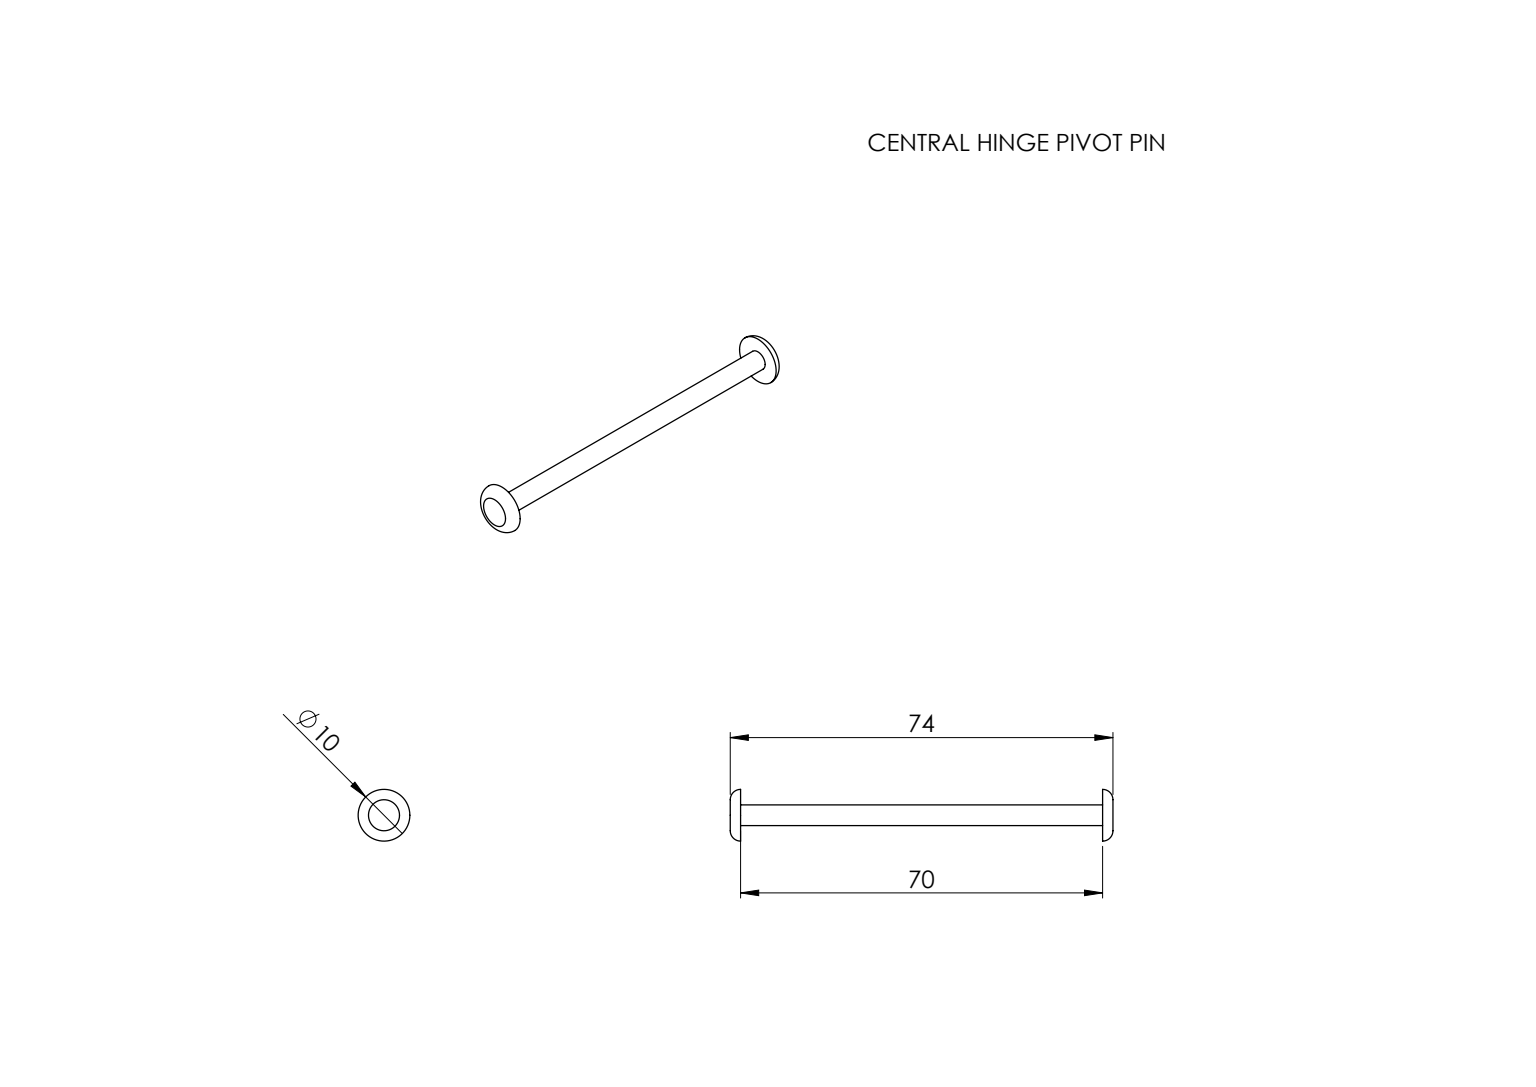
ISO-10303-21;
HEADER;
FILE_DESCRIPTION (('STEP AP214'),
    '1' );
FILE_NAME ('Central Hinge Pivot Pin.step',
    '2026-10-02T13:02:33',
    ( '' ),
    ( '' ),
    'SwSTEP 2.0',
    'SolidWorks 2026',
    '' );
FILE_SCHEMA (( 'AUTOMOTIVE_DESIGN' ));
ENDSEC;

DATA;
#71=CIRCLE ( 'NONE', #9451, 3.000000000000000000 ) ;
#84=CARTESIAN_POINT ( 'NONE',  ( 0.000000000000000000, 0.000000000000000000, 35.00000000000000000 ) ) ;
#87=( GEOMETRIC_REPRESENTATION_CONTEXT ( 3 ) GLOBAL_UNCERTAINTY_ASSIGNED_CONTEXT ( ( #8912 ) ) GLOBAL_UNIT_ASSIGNED_CONTEXT ( ( #3872, #4067, #6666 ) ) REPRESENTATION_CONTEXT ( 'NONE', 'WORKASPACE' ) );
#156=EDGE_LOOP ( 'NONE', ( #2014, #11521, #8711, #17506 ) ) ;
#171=FACE_OUTER_BOUND ( 'NONE', #4320, .T. ) ;
#180=ORIENTED_EDGE ( 'NONE', *, *, #16256, .T. ) ;
#259=DIRECTION ( 'NONE',  ( 1.000000000000000000, 0.000000000000000000, -0.000000000000000000 ) ) ;
#293=DIRECTION ( 'NONE',  ( -1.000000000000000000, 0.000000000000000000, 0.000000000000000000 ) ) ;
#355=CIRCLE ( 'NONE', #13059, 2.000000000000000000 ) ;
#373=ORIENTED_EDGE ( 'NONE', *, *, #11541, .F. ) ;
#379=ORIENTED_EDGE ( 'NONE', *, *, #9515, .T. ) ;
#388=STYLED_ITEM ( 'NONE', ( #17094 ), #8708 ) ;
#454=PRODUCT ( 'Central Hinge Pivot Pin', 'Central Hinge Pivot Pin', '', ( #9983 ) ) ;
#476=CARTESIAN_POINT ( 'NONE',  ( 3.000000000000000000, 4.898587196589412829E-16, -37.00000000000000711 ) ) ;
#676=CARTESIAN_POINT ( 'NONE',  ( 0.000000000000000000, 0.000000000000000000, 35.00000000000000000 ) ) ;
#732=CARTESIAN_POINT ( 'NONE',  ( 0.000000000000000000, 0.000000000000000000, -35.00000000000000000 ) ) ;
#784=SURFACE_SIDE_STYLE ('',( #16717 ) ) ;
#816=DIRECTION ( 'NONE',  ( 0.000000000000000000, 0.000000000000000000, 1.000000000000000000 ) ) ;
#899=DIRECTION ( 'NONE',  ( 0.000000000000000000, 0.000000000000000000, -1.000000000000000000 ) ) ;
#927=ADVANCED_FACE ( 'NONE', ( #17116 ), #14530, .T. ) ;
#967=CIRCLE ( 'NONE', #3346, 2.000000000000001776 ) ;
#1020=DIRECTION ( 'NONE',  ( -0.000000000000000000, -0.000000000000000000, -1.000000000000000000 ) ) ;
#1061=ORIENTED_EDGE ( 'NONE', *, *, #6669, .F. ) ;
#1218=FACE_OUTER_BOUND ( 'NONE', #3277, .T. ) ;
#1275=ORIENTED_EDGE ( 'NONE', *, *, #17968, .T. ) ;
#1295=DIRECTION ( 'NONE',  ( 1.000000000000000000, 0.000000000000000000, 0.000000000000000000 ) ) ;
#1354=CARTESIAN_POINT ( 'NONE',  ( 0.000000000000000000, 0.000000000000000000, -35.00000000000000000 ) ) ;
#1762=DIRECTION ( 'NONE',  ( 1.000000000000000000, 0.000000000000000000, 0.000000000000000000 ) ) ;
#1884=FACE_OUTER_BOUND ( 'NONE', #16108, .T. ) ;
#1930=EDGE_LOOP ( 'NONE', ( #9001, #9036, #2188, #4675 ) ) ;
#1944=PRESENTATION_STYLE_ASSIGNMENT (( #8874 ) ) ;
#1972=EDGE_LOOP ( 'NONE', ( #15195, #7068 ) ) ;
#1996=FACE_OUTER_BOUND ( 'NONE', #18432, .T. ) ;
#2014=ORIENTED_EDGE ( 'NONE', *, *, #11541, .T. ) ;
#2065=DIRECTION ( 'NONE',  ( 1.000000000000000000, 0.000000000000000000, 0.000000000000000000 ) ) ;
#2110=PRODUCT_DEFINITION ( 'UNKNOWN', '', #18444, #16492 ) ;
#2188=ORIENTED_EDGE ( 'NONE', *, *, #15045, .F. ) ;
#2222=DIRECTION ( 'NONE',  ( 1.000000000000000000, 0.000000000000000000, 0.000000000000000000 ) ) ;
#2273=ORIENTED_EDGE ( 'NONE', *, *, #3881, .T. ) ;
#2347=ORIENTED_EDGE ( 'NONE', *, *, #17236, .F. ) ;
#2378=TOROIDAL_SURFACE ( 'NONE', #5096, 3.000000000000000000, 2.000000000000000000 ) ;
#2422=CIRCLE ( 'NONE', #13007, 5.000000000000000000 ) ;
#2462=EDGE_CURVE ( 'NONE', #8941, #8532, #71, .T. ) ;
#2485=LINE ( 'NONE', #15360, #17967 ) ;
#2610=DIRECTION ( 'NONE',  ( 1.000000000000000000, 0.000000000000000000, 0.000000000000000000 ) ) ;
#2638=FACE_OUTER_BOUND ( 'NONE', #10893, .T. ) ;
#2654=VERTEX_POINT ( 'NONE', #9678 ) ;
#2742=DIRECTION ( 'NONE',  ( 0.000000000000000000, 0.000000000000000000, 1.000000000000000000 ) ) ;
#2755=DIRECTION ( 'NONE',  ( 0.000000000000000000, 0.000000000000000000, 1.000000000000000000 ) ) ;
#3019=ADVANCED_FACE ( 'NONE', ( #4031 ), #15601, .T. ) ;
#3081=FILL_AREA_STYLE_COLOUR ( '', #13822 ) ;
#3129=DIRECTION ( 'NONE',  ( -1.000000000000000000, 0.000000000000000000, 0.000000000000000000 ) ) ;
#3253=( NAMED_UNIT ( * ) PLANE_ANGLE_UNIT ( ) SI_UNIT ( $, .RADIAN. ) );
#3271=CIRCLE ( 'NONE', #10551, 3.000000000000000000 ) ;
#3277=EDGE_LOOP ( 'NONE', ( #2347, #7274, #18296, #12313 ) ) ;
#3346=AXIS2_PLACEMENT_3D ( 'NONE', #12462, #6513, #8306 ) ;
#3434=ADVANCED_FACE ( 'NONE', ( #7901 ), #10506, .T. ) ;
#3547=DIRECTION ( 'NONE',  ( 0.000000000000000000, 0.000000000000000000, -1.000000000000000000 ) ) ;
#3744=DIRECTION ( 'NONE',  ( 0.000000000000000000, 0.000000000000000000, 1.000000000000000000 ) ) ;
#3838=VERTEX_POINT ( 'NONE', #9282 ) ;
#3872=( LENGTH_UNIT ( ) NAMED_UNIT ( * ) SI_UNIT ( .MILLI., .METRE. ) );
#3874=CIRCLE ( 'NONE', #16614, 2.000000000000000000 ) ;
#3881=EDGE_CURVE ( 'NONE', #10603, #16711, #2422, .T. ) ;
#3973=DIRECTION ( 'NONE',  ( 1.000000000000000000, 0.000000000000000000, 0.000000000000000000 ) ) ;
#4031=FACE_OUTER_BOUND ( 'NONE', #14769, .T. ) ;
#4036=VERTEX_POINT ( 'NONE', #14821 ) ;
#4067=( NAMED_UNIT ( * ) PLANE_ANGLE_UNIT ( ) SI_UNIT ( $, .RADIAN. ) );
#4096=CARTESIAN_POINT ( 'NONE',  ( 0.000000000000000000, 0.000000000000000000, 35.00000000000000000 ) ) ;
#4141=PLANE ( 'NONE',  #5570 ) ;
#4183=DIRECTION ( 'NONE',  ( -1.000000000000000000, 1.224646799147353207E-16, 0.000000000000000000 ) ) ;
#4256=AXIS2_PLACEMENT_3D ( 'NONE', #732, #8958, #16371 ) ;
#4313=DIRECTION ( 'NONE',  ( 0.000000000000000000, 0.000000000000000000, 1.000000000000000000 ) ) ;
#4320=EDGE_LOOP ( 'NONE', ( #4636, #8294 ) ) ;
#4452=( GEOMETRIC_REPRESENTATION_CONTEXT ( 3 ) GLOBAL_UNCERTAINTY_ASSIGNED_CONTEXT ( ( #5444 ) ) GLOBAL_UNIT_ASSIGNED_CONTEXT ( ( #4502, #6419, #10283 ) ) REPRESENTATION_CONTEXT ( 'NONE', 'WORKASPACE' ) );
#4502=( LENGTH_UNIT ( ) NAMED_UNIT ( * ) SI_UNIT ( .MILLI., .METRE. ) );
#4516=EDGE_CURVE ( 'NONE', #10603, #8941, #8765, .T. ) ;
#4561=DIRECTION ( 'NONE',  ( 0.000000000000000000, 0.000000000000000000, -1.000000000000000000 ) ) ;
#4605=FACE_BOUND ( 'NONE', #1972, .T. ) ;
#4628=ORIENTED_EDGE ( 'NONE', *, *, #9298, .F. ) ;
#4636=ORIENTED_EDGE ( 'NONE', *, *, #8156, .F. ) ;
#4675=ORIENTED_EDGE ( 'NONE', *, *, #16432, .F. ) ;
#4681=ORIENTED_EDGE ( 'NONE', *, *, #10044, .F. ) ;
#4787=AXIS2_PLACEMENT_3D ( 'NONE', #15207, #1020, #2222 ) ;
#4803=ADVANCED_FACE ( 'NONE', ( #11642 ), #12064, .T. ) ;
#5007=ADVANCED_FACE ( 'NONE', ( #1884 ), #6066, .T. ) ;
#5024=CARTESIAN_POINT ( 'NONE',  ( 5.000000000000000000, 0.000000000000000000, 35.00000000000000000 ) ) ;
#5054=CIRCLE ( 'NONE', #17804, 2.000000000000000000 ) ;
#5071=CARTESIAN_POINT ( 'NONE',  ( 0.000000000000000000, 0.000000000000000000, -35.00000000000000000 ) ) ;
#5096=AXIS2_PLACEMENT_3D ( 'NONE', #7416, #10519, #6283 ) ;
#5163=CIRCLE ( 'NONE', #18227, 5.000000000000000000 ) ;
#5180=EDGE_LOOP ( 'NONE', ( #373, #17700 ) ) ;
#5261=CIRCLE ( 'NONE', #10986, 2.000000000000001776 ) ;
#5373=CARTESIAN_POINT ( 'NONE',  ( -3.000000000000000000, 0.000000000000000000, -37.00000000000000711 ) ) ;
#5444=UNCERTAINTY_MEASURE_WITH_UNIT (LENGTH_MEASURE( 1.000000000000000082E-05 ), #4502, 'distance_accuracy_value', 'NONE');
#5447=AXIS2_PLACEMENT_3D ( 'NONE', #4096, #8485, #1295 ) ;
#5570=AXIS2_PLACEMENT_3D ( 'NONE', #18529, #17077, #9846 ) ;
#5766=DIRECTION ( 'NONE',  ( -1.224646799147353207E-16, 1.000000000000000000, 0.000000000000000000 ) ) ;
#5851=DIRECTION ( 'NONE',  ( -1.000000000000000000, -1.224646799147353207E-16, 0.000000000000000000 ) ) ;
#5887=DIRECTION ( 'NONE',  ( -0.000000000000000000, -0.000000000000000000, -1.000000000000000000 ) ) ;
#5951=DIRECTION ( 'NONE',  ( 0.000000000000000000, 0.000000000000000000, 1.000000000000000000 ) ) ;
#6029=CLOSED_SHELL ( 'NONE', ( #3434, #4803, #5007, #7101, #3019, #9319, #9262, #16192, #17067, #927 ) ) ;
#6066=CYLINDRICAL_SURFACE ( 'NONE', #18164, 2.000000000000000000 ) ;
#6198=VERTEX_POINT ( 'NONE', #15959 ) ;
#6246=VERTEX_POINT ( 'NONE', #10038 ) ;
#6283=DIRECTION ( 'NONE',  ( -1.000000000000000000, 0.000000000000000000, 0.000000000000000000 ) ) ;
#6307=ORIENTED_EDGE ( 'NONE', *, *, #4516, .F. ) ;
#6419=( NAMED_UNIT ( * ) PLANE_ANGLE_UNIT ( ) SI_UNIT ( $, .RADIAN. ) );
#6513=DIRECTION ( 'NONE',  ( 0.000000000000000000, -1.000000000000000000, 0.000000000000000000 ) ) ;
#6666=( NAMED_UNIT ( * ) SI_UNIT ( $, .STERADIAN. ) SOLID_ANGLE_UNIT ( ) );
#6669=EDGE_CURVE ( 'NONE', #7437, #4036, #13199, .T. ) ;
#6721=DIRECTION ( 'NONE',  ( 0.000000000000000000, 0.000000000000000000, -1.000000000000000000 ) ) ;
#6821=ORIENTED_EDGE ( 'NONE', *, *, #16993, .F. ) ;
#6967=DIRECTION ( 'NONE',  ( 1.224646799147353207E-16, 1.000000000000000000, -0.000000000000000000 ) ) ;
#7068=ORIENTED_EDGE ( 'NONE', *, *, #6669, .T. ) ;
#7101=ADVANCED_FACE ( 'NONE', ( #1218 ), #11226, .T. ) ;
#7146=CARTESIAN_POINT ( 'NONE',  ( 0.000000000000000000, 0.000000000000000000, -35.00000000000000000 ) ) ;
#7274=ORIENTED_EDGE ( 'NONE', *, *, #11042, .F. ) ;
#7416=CARTESIAN_POINT ( 'NONE',  ( 0.000000000000000000, 0.000000000000000000, -35.00000000000000000 ) ) ;
#7437=VERTEX_POINT ( 'NONE', #9607 ) ;
#7451=FILL_AREA_STYLE ('',( #3081 ) ) ;
#7469=FACE_BOUND ( 'NONE', #13105, .T. ) ;
#7473=DIRECTION ( 'NONE',  ( 0.000000000000000000, 0.000000000000000000, 1.000000000000000000 ) ) ;
#7496=MECHANICAL_DESIGN_GEOMETRIC_PRESENTATION_REPRESENTATION('',(#16262),#18733);
#7542=( NAMED_UNIT ( * ) SI_UNIT ( $, .STERADIAN. ) SOLID_ANGLE_UNIT ( ) );
#7646=SURFACE_STYLE_FILL_AREA ( #7451 ) ;
#7728=SHAPE_REPRESENTATION_RELATIONSHIP ( 'NONE' , 'NONE' ,  #13127, #14079 ) ;
#7901=FACE_OUTER_BOUND ( 'NONE', #1930, .T. ) ;
#8156=EDGE_CURVE ( 'NONE', #13974, #2654, #14279, .T. ) ;
#8163=AXIS2_PLACEMENT_3D ( 'NONE', #11505, #5766, #5851 ) ;
#8274=SURFACE_STYLE_USAGE ( .BOTH. , #784 ) ;
#8294=ORIENTED_EDGE ( 'NONE', *, *, #16256, .F. ) ;
#8306=DIRECTION ( 'NONE',  ( 0.000000000000000000, 0.000000000000000000, -1.000000000000000000 ) ) ;
#8485=DIRECTION ( 'NONE',  ( 0.000000000000000000, 0.000000000000000000, 1.000000000000000000 ) ) ;
#8532=VERTEX_POINT ( 'NONE', #5373 ) ;
#8535=DIRECTION ( 'NONE',  ( 1.000000000000000000, 0.000000000000000000, 0.000000000000000000 ) ) ;
#8591=AXIS2_PLACEMENT_3D ( 'NONE', #15717, #2742, #8535 ) ;
#8696=EDGE_CURVE ( 'NONE', #4036, #3838, #2485, .T. ) ;
#8708=MANIFOLD_SOLID_BREP ( 'Fillet1', #6029 ) ;
#8711=ORIENTED_EDGE ( 'NONE', *, *, #16898, .F. ) ;
#8765=CIRCLE ( 'NONE', #8163, 2.000000000000000000 ) ;
#8792=DIRECTION ( 'NONE',  ( 1.000000000000000000, 0.000000000000000000, 0.000000000000000000 ) ) ;
#8874=SURFACE_STYLE_USAGE ( .BOTH. , #13583 ) ;
#8912=UNCERTAINTY_MEASURE_WITH_UNIT (LENGTH_MEASURE( 1.000000000000000082E-05 ), #3872, 'distance_accuracy_value', 'NONE');
#8941=VERTEX_POINT ( 'NONE', #476 ) ;
#8958=DIRECTION ( 'NONE',  ( 0.000000000000000000, 0.000000000000000000, -1.000000000000000000 ) ) ;
#9001=ORIENTED_EDGE ( 'NONE', *, *, #8156, .T. ) ;
#9036=ORIENTED_EDGE ( 'NONE', *, *, #16993, .T. ) ;
#9262=ADVANCED_FACE ( 'NONE', ( #2638 ), #4141, .T. ) ;
#9282=CARTESIAN_POINT ( 'NONE',  ( 2.000000000000000000, 0.000000000000000000, 35.00000000000000000 ) ) ;
#9298=EDGE_CURVE ( 'NONE', #13520, #6246, #15842, .T. ) ;
#9319=ADVANCED_FACE ( 'NONE', ( #7469, #171 ), #10581, .F. ) ;
#9395=DIRECTION ( 'NONE',  ( 0.000000000000000000, 0.000000000000000000, 1.000000000000000000 ) ) ;
#9451=AXIS2_PLACEMENT_3D ( 'NONE', #13259, #10141, #293 ) ;
#9515=EDGE_CURVE ( 'NONE', #16711, #8532, #5261, .T. ) ;
#9582=DIRECTION ( 'NONE',  ( 0.000000000000000000, 0.000000000000000000, 1.000000000000000000 ) ) ;
#9607=CARTESIAN_POINT ( 'NONE',  ( -2.000000000000000000, 2.449293598294706414E-16, -35.00000000000000000 ) ) ;
#9612=AXIS2_PLACEMENT_3D ( 'NONE', #15732, #2755, #14113 ) ;
#9678=CARTESIAN_POINT ( 'NONE',  ( -5.000000000000000000, 6.123233995736766282E-16, 35.00000000000000000 ) ) ;
#9819=DIRECTION ( 'NONE',  ( 0.000000000000000000, 0.000000000000000000, 1.000000000000000000 ) ) ;
#9842=ORIENTED_EDGE ( 'NONE', *, *, #2462, .T. ) ;
#9846=DIRECTION ( 'NONE',  ( -1.000000000000000000, 0.000000000000000000, -0.000000000000000000 ) ) ;
#9983=PRODUCT_CONTEXT ( 'NONE', #12312, 'mechanical' ) ;
#10038=CARTESIAN_POINT ( 'NONE',  ( 3.000000000000000000, 0.000000000000000000, 37.00000000000000711 ) ) ;
#10044=EDGE_CURVE ( 'NONE', #3838, #6198, #355, .T. ) ;
#10076=ORIENTED_EDGE ( 'NONE', *, *, #10044, .T. ) ;
#10089=DIRECTION ( 'NONE',  ( 1.000000000000000000, 0.000000000000000000, 0.000000000000000000 ) ) ;
#10125=EDGE_LOOP ( 'NONE', ( #6821, #180, #11340, #4628 ) ) ;
#10141=DIRECTION ( 'NONE',  ( 0.000000000000000000, 0.000000000000000000, -1.000000000000000000 ) ) ;
#10283=( NAMED_UNIT ( * ) SI_UNIT ( $, .STERADIAN. ) SOLID_ANGLE_UNIT ( ) );
#10387=APPLICATION_CONTEXT ( 'automotive_design' ) ;
#10506=TOROIDAL_SURFACE ( 'NONE', #9612, 3.000000000000000000, 2.000000000000000000 ) ;
#10519=DIRECTION ( 'NONE',  ( 0.000000000000000000, 0.000000000000000000, -1.000000000000000000 ) ) ;
#10551=AXIS2_PLACEMENT_3D ( 'NONE', #18171, #899, #10909 ) ;
#10581=PLANE ( 'NONE',  #14333 ) ;
#10589=ORIENTED_EDGE ( 'NONE', *, *, #2462, .F. ) ;
#10603=VERTEX_POINT ( 'NONE', #11237 ) ;
#10623=ORIENTED_EDGE ( 'NONE', *, *, #15045, .T. ) ;
#10685=CARTESIAN_POINT ( 'NONE',  ( 0.000000000000000000, 0.000000000000000000, -40.65685424949239035 ) ) ;
#10696=DIRECTION ( 'NONE',  ( 1.000000000000000000, 0.000000000000000000, 0.000000000000000000 ) ) ;
#10893=EDGE_LOOP ( 'NONE', ( #15015, #9842 ) ) ;
#10909=DIRECTION ( 'NONE',  ( -1.000000000000000000, 0.000000000000000000, 0.000000000000000000 ) ) ;
#10954=MECHANICAL_DESIGN_GEOMETRIC_PRESENTATION_REPRESENTATION('',(#388),#87);
#10986=AXIS2_PLACEMENT_3D ( 'NONE', #12176, #16776, #6721 ) ;
#11042=EDGE_CURVE ( 'NONE', #4036, #7437, #13547, .T. ) ;
#11111=CARTESIAN_POINT ( 'NONE',  ( 0.000000000000000000, 0.000000000000000000, 37.00000000000000711 ) ) ;
#11226=CYLINDRICAL_SURFACE ( 'NONE', #13639, 2.000000000000000000 ) ;
#11237=CARTESIAN_POINT ( 'NONE',  ( 5.000000000000000000, 6.123233995736766282E-16, -35.00000000000000000 ) ) ;
#11260=CARTESIAN_POINT ( 'NONE',  ( 0.000000000000000000, 0.000000000000000000, -35.00000000000000000 ) ) ;
#11340=ORIENTED_EDGE ( 'NONE', *, *, #16432, .T. ) ;
#11360=ORIENTED_EDGE ( 'NONE', *, *, #9298, .T. ) ;
#11505=CARTESIAN_POINT ( 'NONE',  ( 3.000000000000000000, 3.673940397442059868E-16, -35.00000000000000000 ) ) ;
#11521=ORIENTED_EDGE ( 'NONE', *, *, #4516, .T. ) ;
#11541=EDGE_CURVE ( 'NONE', #16711, #10603, #12354, .T. ) ;
#11582=SHAPE_DEFINITION_REPRESENTATION ( #16837, #13127 ) ;
#11642=FACE_OUTER_BOUND ( 'NONE', #156, .T. ) ;
#11674=AXIS2_PLACEMENT_3D ( 'NONE', #18514, #3744, #18415 ) ;
#11956=CARTESIAN_POINT ( 'NONE',  ( -3.000000000000000000, 4.898587196589412829E-16, 37.00000000000000711 ) ) ;
#12029=AXIS2_PLACEMENT_3D ( 'NONE', #11260, #18342, #14018 ) ;
#12040=CARTESIAN_POINT ( 'NONE',  ( -5.000000000000000000, 0.000000000000000000, -35.00000000000000000 ) ) ;
#12064=TOROIDAL_SURFACE ( 'NONE', #14523, 3.000000000000000000, 2.000000000000000000 ) ;
#12176=CARTESIAN_POINT ( 'NONE',  ( -3.000000000000000000, 0.000000000000000000, -35.00000000000000000 ) ) ;
#12202=ORIENTED_EDGE ( 'NONE', *, *, #8696, .F. ) ;
#12206=LINE ( 'NONE', #18144, #13891 ) ;
#12312=APPLICATION_CONTEXT ( 'automotive_design' ) ;
#12313=ORIENTED_EDGE ( 'NONE', *, *, #17968, .F. ) ;
#12354=CIRCLE ( 'NONE', #12029, 5.000000000000000000 ) ;
#12367=DIRECTION ( 'NONE',  ( -1.000000000000000000, 0.000000000000000000, 0.000000000000000000 ) ) ;
#12420=FILL_AREA_STYLE_COLOUR ( '', #16134 ) ;
#12462=CARTESIAN_POINT ( 'NONE',  ( 3.000000000000000000, 0.000000000000000000, 35.00000000000000000 ) ) ;
#12597=FILL_AREA_STYLE ('',( #12420 ) ) ;
#12902=AXIS2_PLACEMENT_3D ( 'NONE', #11111, #816, #16541 ) ;
#13007=AXIS2_PLACEMENT_3D ( 'NONE', #5071, #3547, #12367 ) ;
#13059=AXIS2_PLACEMENT_3D ( 'NONE', #676, #17947, #10696 ) ;
#13105=EDGE_LOOP ( 'NONE', ( #10076, #1275 ) ) ;
#13127=SHAPE_REPRESENTATION ( 'Central Hinge Pivot Pin', ( #18772 ), #4452 ) ;
#13199=CIRCLE ( 'NONE', #13781, 2.000000000000000000 ) ;
#13259=CARTESIAN_POINT ( 'NONE',  ( 0.000000000000000000, 0.000000000000000000, -37.00000000000000711 ) ) ;
#13406=PLANE ( 'NONE',  #4256 ) ;
#13503=CIRCLE ( 'NONE', #12902, 3.000000000000000000 ) ;
#13520=VERTEX_POINT ( 'NONE', #11956 ) ;
#13547=CIRCLE ( 'NONE', #4787, 2.000000000000000000 ) ;
#13583=SURFACE_SIDE_STYLE ('',( #7646 ) ) ;
#13593=DIRECTION ( 'NONE',  ( 0.000000000000000000, 0.000000000000000000, 1.000000000000000000 ) ) ;
#13611=CARTESIAN_POINT ( 'NONE',  ( 0.000000000000000000, 0.000000000000000000, 0.000000000000000000 ) ) ;
#13639=AXIS2_PLACEMENT_3D ( 'NONE', #17049, #9819, #2610 ) ;
#13686=FACE_OUTER_BOUND ( 'NONE', #5180, .T. ) ;
#13781=AXIS2_PLACEMENT_3D ( 'NONE', #1354, #5887, #3973 ) ;
#13822=COLOUR_RGB ( '', 0.72549020, 0.75294118, 0.79215686) ;
#13891=VECTOR ( 'NONE', #9395, 1000.000000000000000 ) ;
#13974=VERTEX_POINT ( 'NONE', #5024 ) ;
#14018=DIRECTION ( 'NONE',  ( -1.000000000000000000, 0.000000000000000000, 0.000000000000000000 ) ) ;
#14079=ADVANCED_BREP_SHAPE_REPRESENTATION ( '', ( #8708, #18772 ), #4452 ) ;
#14113=DIRECTION ( 'NONE',  ( 1.000000000000000000, 0.000000000000000000, 0.000000000000000000 ) ) ;
#14143=CARTESIAN_POINT ( 'NONE',  ( -3.000000000000000000, 3.673940397442059868E-16, 35.00000000000000000 ) ) ;
#14186=ORIENTED_EDGE ( 'NONE', *, *, #17236, .T. ) ;
#14279=CIRCLE ( 'NONE', #15789, 5.000000000000000000 ) ;
#14333=AXIS2_PLACEMENT_3D ( 'NONE', #16474, #5951, #259 ) ;
#14523=AXIS2_PLACEMENT_3D ( 'NONE', #7146, #4561, #3129 ) ;
#14530=TOROIDAL_SURFACE ( 'NONE', #5447, 3.000000000000000000, 2.000000000000000000 ) ;
#14745=CARTESIAN_POINT ( 'NONE',  ( 0.000000000000000000, 0.000000000000000000, 35.00000000000000000 ) ) ;
#14759=DIRECTION ( 'NONE',  ( 1.000000000000000000, 0.000000000000000000, 0.000000000000000000 ) ) ;
#14769=EDGE_LOOP ( 'NONE', ( #10623, #11360 ) ) ;
#14821=CARTESIAN_POINT ( 'NONE',  ( 2.000000000000000000, 0.000000000000000000, -35.00000000000000000 ) ) ;
#14953=DIRECTION ( 'NONE',  ( 0.000000000000000000, 0.000000000000000000, 1.000000000000000000 ) ) ;
#15015=ORIENTED_EDGE ( 'NONE', *, *, #16898, .T. ) ;
#15045=EDGE_CURVE ( 'NONE', #6246, #13520, #13503, .T. ) ;
#15195=ORIENTED_EDGE ( 'NONE', *, *, #11042, .T. ) ;
#15207=CARTESIAN_POINT ( 'NONE',  ( 0.000000000000000000, 0.000000000000000000, -35.00000000000000000 ) ) ;
#15360=CARTESIAN_POINT ( 'NONE',  ( 2.000000000000000000, 0.000000000000000000, -40.65685424949239035 ) ) ;
#15601=PLANE ( 'NONE',  #11674 ) ;
#15717=CARTESIAN_POINT ( 'NONE',  ( 0.000000000000000000, 0.000000000000000000, 37.00000000000000711 ) ) ;
#15732=CARTESIAN_POINT ( 'NONE',  ( 0.000000000000000000, 0.000000000000000000, 35.00000000000000000 ) ) ;
#15789=AXIS2_PLACEMENT_3D ( 'NONE', #84, #18622, #8792 ) ;
#15842=CIRCLE ( 'NONE', #8591, 3.000000000000000000 ) ;
#15959=CARTESIAN_POINT ( 'NONE',  ( -2.000000000000000000, 2.449293598294706414E-16, 35.00000000000000000 ) ) ;
#16108=EDGE_LOOP ( 'NONE', ( #1061, #14186, #4681, #12202 ) ) ;
#16134=COLOUR_RGB ( '', 0.72549020, 0.75294118, 0.79215686) ;
#16173=( LENGTH_UNIT ( ) NAMED_UNIT ( * ) SI_UNIT ( .MILLI., .METRE. ) );
#16192=ADVANCED_FACE ( 'NONE', ( #4605, #13686 ), #13406, .F. ) ;
#16256=EDGE_CURVE ( 'NONE', #2654, #13974, #5163, .T. ) ;
#16262=STYLED_ITEM ( 'NONE', ( #1944 ), #14079 ) ;
#16371=DIRECTION ( 'NONE',  ( -1.000000000000000000, 0.000000000000000000, -0.000000000000000000 ) ) ;
#16432=EDGE_CURVE ( 'NONE', #13974, #6246, #967, .T. ) ;
#16474=CARTESIAN_POINT ( 'NONE',  ( 0.000000000000000000, 0.000000000000000000, 35.00000000000000000 ) ) ;
#16492=PRODUCT_DEFINITION_CONTEXT ( 'detailed design', #10387, 'design' ) ;
#16541=DIRECTION ( 'NONE',  ( 1.000000000000000000, 0.000000000000000000, 0.000000000000000000 ) ) ;
#16614=AXIS2_PLACEMENT_3D ( 'NONE', #14143, #6967, #4183 ) ;
#16711=VERTEX_POINT ( 'NONE', #12040 ) ;
#16717=SURFACE_STYLE_FILL_AREA ( #12597 ) ;
#16776=DIRECTION ( 'NONE',  ( -0.000000000000000000, -1.000000000000000000, -0.000000000000000000 ) ) ;
#16837=PRODUCT_DEFINITION_SHAPE ( 'NONE', 'NONE',  #2110 ) ;
#16898=EDGE_CURVE ( 'NONE', #8532, #8941, #3271, .T. ) ;
#16993=EDGE_CURVE ( 'NONE', #2654, #13520, #3874, .T. ) ;
#17032=UNCERTAINTY_MEASURE_WITH_UNIT (LENGTH_MEASURE( 1.000000000000000082E-05 ), #16173, 'distance_accuracy_value', 'NONE');
#17049=CARTESIAN_POINT ( 'NONE',  ( 0.000000000000000000, 0.000000000000000000, -40.65685424949239035 ) ) ;
#17067=ADVANCED_FACE ( 'NONE', ( #1996 ), #2378, .T. ) ;
#17077=DIRECTION ( 'NONE',  ( 0.000000000000000000, 0.000000000000000000, -1.000000000000000000 ) ) ;
#17094=PRESENTATION_STYLE_ASSIGNMENT (( #8274 ) ) ;
#17116=FACE_OUTER_BOUND ( 'NONE', #10125, .T. ) ;
#17236=EDGE_CURVE ( 'NONE', #7437, #6198, #12206, .T. ) ;
#17330=CARTESIAN_POINT ( 'NONE',  ( 0.000000000000000000, 0.000000000000000000, 35.00000000000000000 ) ) ;
#17506=ORIENTED_EDGE ( 'NONE', *, *, #9515, .F. ) ;
#17700=ORIENTED_EDGE ( 'NONE', *, *, #3881, .F. ) ;
#17804=AXIS2_PLACEMENT_3D ( 'NONE', #17330, #4313, #10089 ) ;
#17947=DIRECTION ( 'NONE',  ( 0.000000000000000000, 0.000000000000000000, 1.000000000000000000 ) ) ;
#17967=VECTOR ( 'NONE', #9582, 1000.000000000000000 ) ;
#17968=EDGE_CURVE ( 'NONE', #6198, #3838, #5054, .T. ) ;
#18144=CARTESIAN_POINT ( 'NONE',  ( -2.000000000000000000, 2.449293598294706414E-16, -40.65685424949239035 ) ) ;
#18164=AXIS2_PLACEMENT_3D ( 'NONE', #10685, #14953, #2065 ) ;
#18171=CARTESIAN_POINT ( 'NONE',  ( 0.000000000000000000, 0.000000000000000000, -37.00000000000000711 ) ) ;
#18227=AXIS2_PLACEMENT_3D ( 'NONE', #14745, #13593, #1762 ) ;
#18296=ORIENTED_EDGE ( 'NONE', *, *, #8696, .T. ) ;
#18342=DIRECTION ( 'NONE',  ( 0.000000000000000000, 0.000000000000000000, -1.000000000000000000 ) ) ;
#18415=DIRECTION ( 'NONE',  ( 1.000000000000000000, 0.000000000000000000, -0.000000000000000000 ) ) ;
#18432=EDGE_LOOP ( 'NONE', ( #6307, #2273, #379, #10589 ) ) ;
#18444=PRODUCT_DEFINITION_FORMATION_WITH_SPECIFIED_SOURCE ( 'ANY', '', #454, .NOT_KNOWN. ) ;
#18514=CARTESIAN_POINT ( 'NONE',  ( 0.000000000000000000, 0.000000000000000000, 37.00000000000000711 ) ) ;
#18529=CARTESIAN_POINT ( 'NONE',  ( 0.000000000000000000, 0.000000000000000000, -37.00000000000000711 ) ) ;
#18622=DIRECTION ( 'NONE',  ( 0.000000000000000000, 0.000000000000000000, 1.000000000000000000 ) ) ;
#18733=( GEOMETRIC_REPRESENTATION_CONTEXT ( 3 ) GLOBAL_UNCERTAINTY_ASSIGNED_CONTEXT ( ( #17032 ) ) GLOBAL_UNIT_ASSIGNED_CONTEXT ( ( #16173, #3253, #7542 ) ) REPRESENTATION_CONTEXT ( 'NONE', 'WORKASPACE' ) );
#18772=AXIS2_PLACEMENT_3D ( 'NONE', #13611, #7473, #14759 ) ;
ENDSEC;
END-ISO-10303-21;
